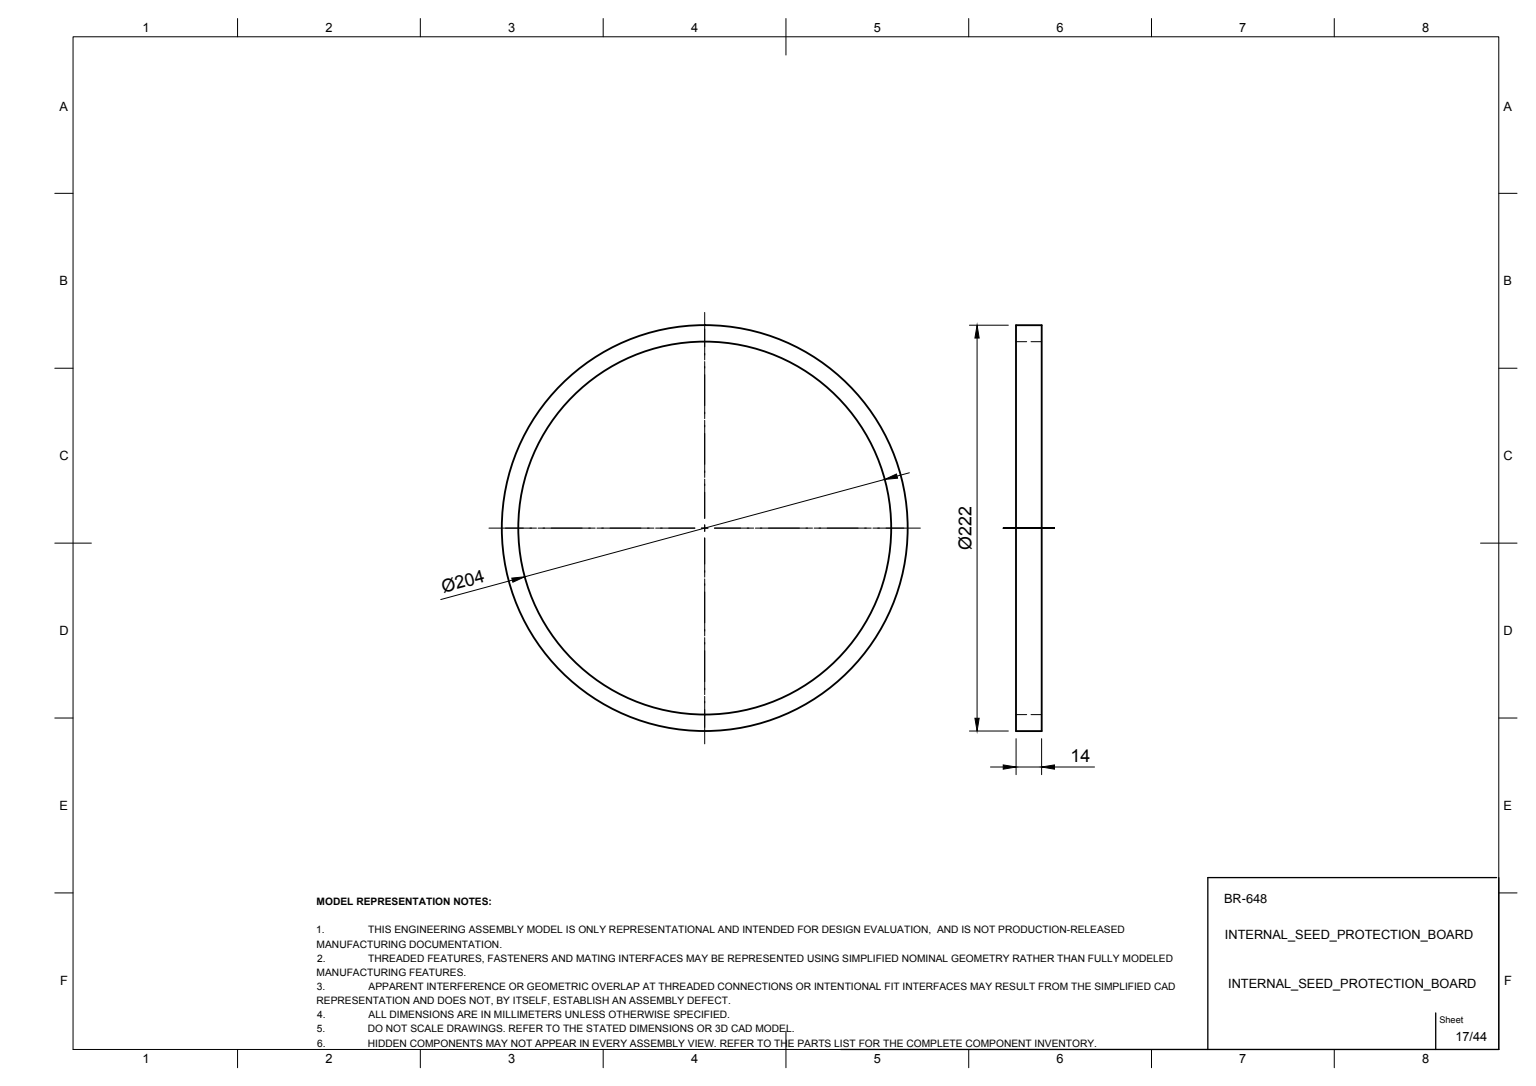
ISO-10303-21;
HEADER;
FILE_DESCRIPTION((''),'2;1');
FILE_NAME('INTERNAL_SEED_PROTECTION_BOARD.step','2026-10-01T22:05:39-07:00',(''),(''),'','','');
FILE_SCHEMA (('AUTOMOTIVE_DESIGN { 1 0 10303 214 3 1 1 }'));
ENDSEC;
DATA;
#10=MECHANICAL_DESIGN_GEOMETRIC_PRESENTATION_REPRESENTATION('',(#617),#24628);
#533=SHAPE_REPRESENTATION_RELATIONSHIP('SRR','None',#24805,#575) ;
#575=ADVANCED_BREP_SHAPE_REPRESENTATION('',(#657),#24595) ;
#617=STYLED_ITEM('',(#25035),#657) ;
#657=MANIFOLD_SOLID_BREP('INTERNAL_SEED_PROTECTION_BOARD',#13128) ;
#852=FACE_BOUND('',#4148,.T.) ;
#853=FACE_BOUND('',#4150,.T.) ;
#1303=LINE('',#21063,#2139) ;
#1304=LINE('',#21069,#2140) ;
#2139=VECTOR('',#16808,10.2) ;
#2140=VECTOR('',#16815,11.1) ;
#2804=CYLINDRICAL_SURFACE('',#14208,10.2) ;
#2805=CYLINDRICAL_SURFACE('',#14211,11.1) ;
#3212=FACE_OUTER_BOUND('',#4145,.T.) ;
#3213=FACE_OUTER_BOUND('',#4146,.T.) ;
#3214=FACE_OUTER_BOUND('',#4147,.T.) ;
#3215=FACE_OUTER_BOUND('',#4149,.T.) ;
#4145=EDGE_LOOP('',(#9663,#9664,#9665,#9666)) ;
#4146=EDGE_LOOP('',(#9667,#9668,#9669,#9670)) ;
#4147=EDGE_LOOP('',(#9671)) ;
#4148=EDGE_LOOP('',(#9672)) ;
#4149=EDGE_LOOP('',(#9673)) ;
#4150=EDGE_LOOP('',(#9674)) ;
#5032=CIRCLE('',#14209,10.2) ;
#5033=CIRCLE('',#14210,10.2) ;
#5034=CIRCLE('',#14212,11.1) ;
#5035=CIRCLE('',#14213,11.1) ;
#5929=VERTEX_POINT('',#21060) ;
#5930=VERTEX_POINT('',#21062) ;
#5931=VERTEX_POINT('',#21066) ;
#5932=VERTEX_POINT('',#21068) ;
#7321=EDGE_CURVE('',#5929,#5929,#5032,.T.) ;
#7322=EDGE_CURVE('',#5929,#5930,#1303,.T.) ;
#7323=EDGE_CURVE('',#5930,#5930,#5033,.T.) ;
#7324=EDGE_CURVE('',#5931,#5931,#5034,.T.) ;
#7325=EDGE_CURVE('',#5931,#5932,#1304,.T.) ;
#7326=EDGE_CURVE('',#5932,#5932,#5035,.T.) ;
#9663=ORIENTED_EDGE('',*,*,#7321,.F.) ;
#9664=ORIENTED_EDGE('',*,*,#7322,.T.) ;
#9665=ORIENTED_EDGE('',*,*,#7323,.F.) ;
#9666=ORIENTED_EDGE('',*,*,#7322,.F.) ;
#9667=ORIENTED_EDGE('',*,*,#7324,.F.) ;
#9668=ORIENTED_EDGE('',*,*,#7325,.T.) ;
#9669=ORIENTED_EDGE('',*,*,#7326,.F.) ;
#9670=ORIENTED_EDGE('',*,*,#7325,.F.) ;
#9671=ORIENTED_EDGE('',*,*,#7326,.T.) ;
#9672=ORIENTED_EDGE('',*,*,#7321,.T.) ;
#9673=ORIENTED_EDGE('',*,*,#7324,.T.) ;
#9674=ORIENTED_EDGE('',*,*,#7323,.T.) ;
#12124=PLANE('',#14214) ;
#12125=PLANE('',#14215) ;
#12607=ADVANCED_FACE('',(#3212),#2804,.F.) ;
#12608=ADVANCED_FACE('',(#3213),#2805,.T.) ;
#12609=ADVANCED_FACE('',(#3214,#852),#12124,.T.) ;
#12610=ADVANCED_FACE('',(#3215,#853),#12125,.T.) ;
#13128=CLOSED_SHELL('',(#12607,#12608,#12609,#12610)) ;
#14207=AXIS2_PLACEMENT_3D('',#21058,#16802,#16803) ;
#14208=AXIS2_PLACEMENT_3D('',#21059,#16804,#16805) ;
#14209=AXIS2_PLACEMENT_3D('',#21061,#16806,#16807) ;
#14210=AXIS2_PLACEMENT_3D('',#21064,#16809,#16810) ;
#14211=AXIS2_PLACEMENT_3D('',#21065,#16811,#16812) ;
#14212=AXIS2_PLACEMENT_3D('',#21067,#16813,#16814) ;
#14213=AXIS2_PLACEMENT_3D('',#21070,#16816,#16817) ;
#14214=AXIS2_PLACEMENT_3D('',#21071,#16818,#16819) ;
#14215=AXIS2_PLACEMENT_3D('',#21072,#16820,#16821) ;
#16802=DIRECTION('axis',(0.,0.,1.)) ;
#16803=DIRECTION('refdir',(1.,0.,0.)) ;
#16804=DIRECTION('center_axis',(0.,1.,0.)) ;
#16805=DIRECTION('ref_axis',(1.,0.,0.)) ;
#16806=DIRECTION('center_axis',(0.,1.,0.)) ;
#16807=DIRECTION('ref_axis',(1.,0.,0.)) ;
#16808=DIRECTION('',(0.,1.,0.)) ;
#16809=DIRECTION('center_axis',(0.,-1.,0.)) ;
#16810=DIRECTION('ref_axis',(1.,0.,0.)) ;
#16811=DIRECTION('center_axis',(0.,1.,0.)) ;
#16812=DIRECTION('ref_axis',(1.,0.,0.)) ;
#16813=DIRECTION('center_axis',(0.,1.,0.)) ;
#16814=DIRECTION('ref_axis',(1.,0.,0.)) ;
#16815=DIRECTION('',(0.,-1.,0.)) ;
#16816=DIRECTION('center_axis',(0.,-1.,0.)) ;
#16817=DIRECTION('ref_axis',(1.,0.,0.)) ;
#16818=DIRECTION('center_axis',(0.,-1.,0.)) ;
#16819=DIRECTION('ref_axis',(-1.,0.,0.)) ;
#16820=DIRECTION('center_axis',(0.,1.,0.)) ;
#16821=DIRECTION('ref_axis',(1.,0.,0.)) ;
#21058=CARTESIAN_POINT('',(0.,0.,0.)) ;
#21059=CARTESIAN_POINT('Origin',(0.,-0.7,0.)) ;
#21060=CARTESIAN_POINT('',(-10.2,-1.4,1.2491397351303E-15)) ;
#21061=CARTESIAN_POINT('Origin',(0.,-1.4,0.)) ;
#21062=CARTESIAN_POINT('',(-10.2,0.,-1.2491397351303E-15)) ;
#21063=CARTESIAN_POINT('',(-10.2,-0.7,1.2491397351303E-15)) ;
#21064=CARTESIAN_POINT('Origin',(0.,0.,0.)) ;
#21065=CARTESIAN_POINT('Origin',(0.,-0.7,0.)) ;
#21066=CARTESIAN_POINT('',(-11.1,0.,1.35935794705356E-15)) ;
#21067=CARTESIAN_POINT('Origin',(0.,0.,0.)) ;
#21068=CARTESIAN_POINT('',(-11.1,-1.4,1.35935794705356E-15)) ;
#21069=CARTESIAN_POINT('',(-11.1,-0.7,1.35935794705356E-15)) ;
#21070=CARTESIAN_POINT('Origin',(0.,-1.4,0.)) ;
#21071=CARTESIAN_POINT('Origin',(0.,-1.4,0.)) ;
#21072=CARTESIAN_POINT('Origin',(0.,0.,0.)) ;
#24547=UNCERTAINTY_MEASURE_WITH_UNIT(LENGTH_MEASURE(0.001),#24629,
'DISTANCE_ACCURACY_VALUE',
'Maximum model space distance between geometric entities at asserted c
onnectivities') ;
#24580=UNCERTAINTY_MEASURE_WITH_UNIT(LENGTH_MEASURE(0.001),#24629,
'DISTANCE_ACCURACY_VALUE',
'Maximum model space distance between geometric entities at asserted c
onnectivities') ;
#24595=(
GEOMETRIC_REPRESENTATION_CONTEXT(3)
GLOBAL_UNCERTAINTY_ASSIGNED_CONTEXT((#24547))
GLOBAL_UNIT_ASSIGNED_CONTEXT((#24629,#24631,#24632))
REPRESENTATION_CONTEXT('','3D')
) ;
#24628=(
GEOMETRIC_REPRESENTATION_CONTEXT(3)
GLOBAL_UNCERTAINTY_ASSIGNED_CONTEXT((#24580))
GLOBAL_UNIT_ASSIGNED_CONTEXT((#24629,#24631,#24632))
REPRESENTATION_CONTEXT('','3D')
) ;
#24629=(
LENGTH_UNIT()
NAMED_UNIT(*)
SI_UNIT(.CENTI.,.METRE.)
) ;
#24631=(
NAMED_UNIT(*)
PLANE_ANGLE_UNIT()
SI_UNIT($,.RADIAN.)
) ;
#24632=(
NAMED_UNIT(*)
SI_UNIT($,.STERADIAN.)
SOLID_ANGLE_UNIT()
) ;
#24647=SHAPE_DEFINITION_REPRESENTATION(#24694,#24805) ;
#24694=PRODUCT_DEFINITION_SHAPE('',$,#24853) ;
#24805=SHAPE_REPRESENTATION('',(#14207),#24595) ;
#24838=PRODUCT_DEFINITION_CONTEXT('part definition',#24981,'design') ;
#24853=PRODUCT_DEFINITION('INTERNAL_SEED_PROTECTION_BOARD',
'INTERNAL_SEED_PROTECTION_BOARD',#24900,#24838) ;
#24900=PRODUCT_DEFINITION_FORMATION('',$,#24997) ;
#24981=APPLICATION_CONTEXT(
'Core Data for Automotive Mechanical Design Process') ;
#24982=PRODUCT_CONTEXT('part definition',#24981,'mechanical') ;
#24997=PRODUCT('INTERNAL_SEED_PROTECTION_BOARD',
'INTERNAL_SEED_PROTECTION_BOARD',$,(#24982)) ;
#25035=PRESENTATION_STYLE_ASSIGNMENT((#25045)) ;
#25045=SURFACE_STYLE_USAGE(.BOTH.,#25055) ;
#25055=SURFACE_SIDE_STYLE('',(#25065)) ;
#25065=SURFACE_STYLE_FILL_AREA(#25075) ;
#25075=FILL_AREA_STYLE('ABS (White)',(#25085)) ;
#25085=FILL_AREA_STYLE_COLOUR('ABS (White)',#25095) ;
#25095=COLOUR_RGB('ABS (White)', 0.66274510, 0.83137255, 0.94901961) ;
ENDSEC;
END-ISO-10303-21;
